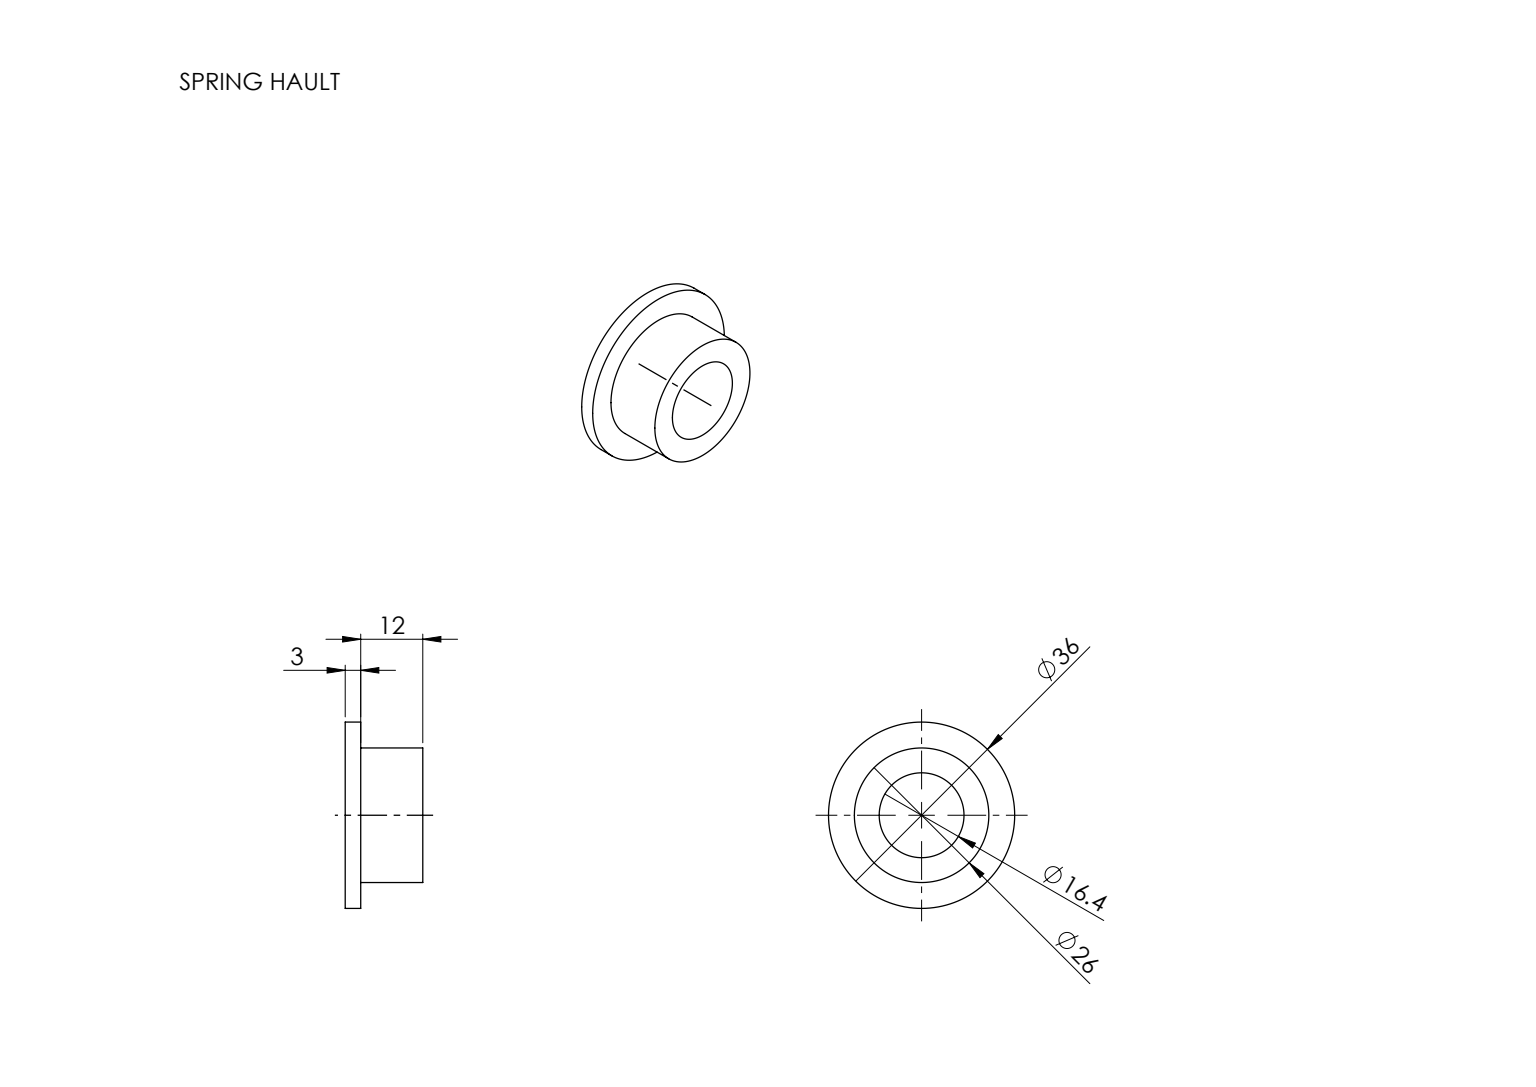
ISO-10303-21;
HEADER;
FILE_DESCRIPTION (('STEP AP214'),
    '1' );
FILE_NAME ('spring hault.step',
    '2026-10-08T13:22:57',
    ( '' ),
    ( '' ),
    'SwSTEP 2.0',
    'SolidWorks 2026',
    '' );
FILE_SCHEMA (( 'AUTOMOTIVE_DESIGN' ));
ENDSEC;

DATA;
#47=CIRCLE ( 'NONE', #69, 13.00000000000001066 ) ;
#65=ORIENTED_EDGE ( 'NONE', *, *, #5817, .F. ) ;
#69=AXIS2_PLACEMENT_3D ( 'NONE', #6608, #9795, #2698 ) ;
#113=( LENGTH_UNIT ( ) NAMED_UNIT ( * ) SI_UNIT ( .MILLI., .METRE. ) );
#143=ORIENTED_EDGE ( 'NONE', *, *, #7111, .T. ) ;
#157=CARTESIAN_POINT ( 'NONE',  ( -58.00000000000002842, 7.703719777548943412E-30, -1.059261469412979719E-30 ) ) ;
#169=CYLINDRICAL_SURFACE ( 'NONE', #4836, 18.00000000000002132 ) ;
#180=CIRCLE ( 'NONE', #1825, 18.00000000000002132 ) ;
#182=ORIENTED_EDGE ( 'NONE', *, *, #837, .T. ) ;
#193=UNCERTAINTY_MEASURE_WITH_UNIT (LENGTH_MEASURE( 1.000000000000000082E-05 ), #7498, 'distance_accuracy_value', 'NONE');
#203=VECTOR ( 'NONE', #8292, 1000.000000000000000 ) ;
#231=EDGE_CURVE ( 'NONE', #1952, #8798, #6117, .T. ) ;
#245=CARTESIAN_POINT ( 'NONE',  ( 0.000000000000000000, 0.000000000000000000, 0.000000000000000000 ) ) ;
#250=ORIENTED_EDGE ( 'NONE', *, *, #8801, .F. ) ;
#286=MANIFOLD_SOLID_BREP ( 'Revolve1', #1357 ) ;
#402=VECTOR ( 'NONE', #5225, 1000.000000000000000 ) ;
#433=EDGE_CURVE ( 'NONE', #9051, #3839, #8410, .T. ) ;
#459=AXIS2_PLACEMENT_3D ( 'NONE', #4903, #3979, #7954 ) ;
#490=CARTESIAN_POINT ( 'NONE',  ( -55.00000000000002132, 7.703719777548943412E-30, -7.703719777548943412E-31 ) ) ;
#571=EDGE_LOOP ( 'NONE', ( #1086, #3200, #2296, #1950 ) ) ;
#603=DIRECTION ( 'NONE',  ( -1.000000000000000000, 1.842239752758738928E-31, -1.780435181894459419E-32 ) ) ;
#626=FACE_OUTER_BOUND ( 'NONE', #2874, .T. ) ;
#649=CARTESIAN_POINT ( 'NONE',  ( -58.00000000000002842, 9.020562075080167263E-17, 13.00000000000001243 ) ) ;
#652=SURFACE_STYLE_FILL_AREA ( #4470 ) ;
#676=ORIENTED_EDGE ( 'NONE', *, *, #3604, .T. ) ;
#694=CYLINDRICAL_SURFACE ( 'NONE', #5832, 18.00000000000002132 ) ;
#707=PLANE ( 'NONE',  #2637 ) ;
#719=ADVANCED_FACE ( 'NONE', ( #7922, #8553 ), #707, .F. ) ;
#752=DIRECTION ( 'NONE',  ( -1.000000000000000000, 1.842239752758738928E-31, -1.780435181894459419E-32 ) ) ;
#795=ORIENTED_EDGE ( 'NONE', *, *, #5893, .F. ) ;
#837=EDGE_CURVE ( 'NONE', #7040, #4031, #8175, .T. ) ;
#849=CIRCLE ( 'NONE', #2646, 8.200000000000009948 ) ;
#863=EDGE_CURVE ( 'NONE', #8514, #4989, #4957, .T. ) ;
#991=FACE_OUTER_BOUND ( 'NONE', #5671, .T. ) ;
#1018=DIRECTION ( 'NONE',  ( 0.000000000000000000, 6.938893903907221444E-18, 1.000000000000000000 ) ) ;
#1021=COLOUR_RGB ( '', 0.72549020, 0.75294118, 0.79215686) ;
#1054=( NAMED_UNIT ( * ) SI_UNIT ( $, .STERADIAN. ) SOLID_ANGLE_UNIT ( ) );
#1073=DIRECTION ( 'NONE',  ( -1.000000000000000000, 1.842239752758738928E-31, -1.780435181894459419E-32 ) ) ;
#1086=ORIENTED_EDGE ( 'NONE', *, *, #4434, .F. ) ;
#1094=CARTESIAN_POINT ( 'NONE',  ( -58.00000000000002132, 5.689893001204698381E-17, 8.200000000000009948 ) ) ;
#1201=DIRECTION ( 'NONE',  ( -1.000000000000000000, 1.842239752758738928E-31, -1.780435181894459419E-32 ) ) ;
#1216=CARTESIAN_POINT ( 'NONE',  ( -43.00000000000002842, 6.933347799794049071E-30, -9.629649721936179265E-31 ) ) ;
#1224=AXIS2_PLACEMENT_3D ( 'NONE', #3055, #7082, #9483 ) ;
#1260=SURFACE_STYLE_USAGE ( .BOTH. , #3745 ) ;
#1297=ORIENTED_EDGE ( 'NONE', *, *, #6791, .F. ) ;
#1357=CLOSED_SHELL ( 'NONE', ( #6188, #6338, #4207, #6354, #4057, #6193, #3933, #5342, #719 ) ) ;
#1452=CARTESIAN_POINT ( 'NONE',  ( -55.00000000000002132, 18.00000000000001776, -1.819825643106760428E-16 ) ) ;
#1516=DIRECTION ( 'NONE',  ( 0.000000000000000000, 6.938893903907221444E-18, 1.000000000000000000 ) ) ;
#1660=EDGE_CURVE ( 'NONE', #7847, #3628, #10060, .T. ) ;
#1770=( NAMED_UNIT ( * ) PLANE_ANGLE_UNIT ( ) SI_UNIT ( $, .RADIAN. ) );
#1825=AXIS2_PLACEMENT_3D ( 'NONE', #3023, #603, #3749 ) ;
#1937=DIRECTION ( 'NONE',  ( -1.000000000000000000, 1.842239752758738928E-31, -1.780435181894459419E-32 ) ) ;
#1950=ORIENTED_EDGE ( 'NONE', *, *, #231, .F. ) ;
#1952=VERTEX_POINT ( 'NONE', #3909 ) ;
#2077=CARTESIAN_POINT ( 'NONE',  ( -58.00000000000002842, 2.079464148194916361E-15, -18.00000000000002132 ) ) ;
#2175=COLOUR_RGB ( '', 0.72549020, 0.75294118, 0.79215686) ;
#2178=PLANE ( 'NONE',  #459 ) ;
#2188=DIRECTION ( 'NONE',  ( -1.000000000000000000, 1.842239752758738928E-31, -1.780435181894459419E-32 ) ) ;
#2205=CARTESIAN_POINT ( 'NONE',  ( -43.00000000000002842, 5.689893001204620728E-17, 8.200000000000009948 ) ) ;
#2296=ORIENTED_EDGE ( 'NONE', *, *, #2974, .T. ) ;
#2301=DIRECTION ( 'NONE',  ( -1.840628461782073167E-32, -6.938893903907220674E-18, -1.000000000000000000 ) ) ;
#2308=ORIENTED_EDGE ( 'NONE', *, *, #5817, .T. ) ;
#2323=CIRCLE ( 'NONE', #9921, 18.00000000000001776 ) ;
#2350=CARTESIAN_POINT ( 'NONE',  ( -43.00000000000002842, 6.933347799794049071E-30, -9.629649721936179265E-31 ) ) ;
#2440=DIRECTION ( 'NONE',  ( 0.000000000000000000, 6.938893903907220674E-18, 1.000000000000000000 ) ) ;
#2478=ORIENTED_EDGE ( 'NONE', *, *, #2974, .F. ) ;
#2491=FILL_AREA_STYLE ('',( #7000 ) ) ;
#2525=DIRECTION ( 'NONE',  ( 0.000000000000000000, 6.938893903907220674E-18, 1.000000000000000000 ) ) ;
#2564=EDGE_CURVE ( 'NONE', #3839, #9051, #9098, .T. ) ;
#2574=ORIENTED_EDGE ( 'NONE', *, *, #4434, .T. ) ;
#2619=ORIENTED_EDGE ( 'NONE', *, *, #863, .F. ) ;
#2629=EDGE_LOOP ( 'NONE', ( #1297, #182, #3115, #7849 ) ) ;
#2637=AXIS2_PLACEMENT_3D ( 'NONE', #6994, #3069, #2301 ) ;
#2646=AXIS2_PLACEMENT_3D ( 'NONE', #1216, #6571, #9806 ) ;
#2698=DIRECTION ( 'NONE',  ( 0.000000000000000000, 6.938893903907221444E-18, 1.000000000000000000 ) ) ;
#2718=ORIENTED_EDGE ( 'NONE', *, *, #1660, .T. ) ;
#2725=PRODUCT_CONTEXT ( 'NONE', #5533, 'mechanical' ) ;
#2742=AXIS2_PLACEMENT_3D ( 'NONE', #7490, #8319, #5061 ) ;
#2808=( NAMED_UNIT ( * ) SI_UNIT ( $, .STERADIAN. ) SOLID_ANGLE_UNIT ( ) );
#2842=AXIS2_PLACEMENT_3D ( 'NONE', #3609, #6028, #9208 ) ;
#2859=( NAMED_UNIT ( * ) PLANE_ANGLE_UNIT ( ) SI_UNIT ( $, .RADIAN. ) );
#2874=EDGE_LOOP ( 'NONE', ( #5790, #7225 ) ) ;
#2883=CARTESIAN_POINT ( 'NONE',  ( -43.00000000000002842, 1.501835218140771832E-15, -13.00000000000000178 ) ) ;
#2974=EDGE_CURVE ( 'NONE', #9051, #8798, #8703, .T. ) ;
#3023=CARTESIAN_POINT ( 'NONE',  ( -58.00000000000002132, 7.703719777548943412E-30, -1.059261469412979719E-30 ) ) ;
#3042=VERTEX_POINT ( 'NONE', #5497 ) ;
#3055=CARTESIAN_POINT ( 'NONE',  ( -58.00000000000002842, 7.703719777548943412E-30, -1.059261469412979719E-30 ) ) ;
#3069=DIRECTION ( 'NONE',  ( 1.000000000000000000, -1.842239752758738928E-31, -1.840628461782073167E-32 ) ) ;
#3115=ORIENTED_EDGE ( 'NONE', *, *, #5908, .T. ) ;
#3165=CARTESIAN_POINT ( 'NONE',  ( -43.00000000000002842, 9.020562075080090842E-17, 13.00000000000001421 ) ) ;
#3200=ORIENTED_EDGE ( 'NONE', *, *, #2564, .T. ) ;
#3211=ORIENTED_EDGE ( 'NONE', *, *, #7111, .F. ) ;
#3221=ORIENTED_EDGE ( 'NONE', *, *, #433, .T. ) ;
#3256=EDGE_LOOP ( 'NONE', ( #10227, #8788, #8586, #3337 ) ) ;
#3259=CARTESIAN_POINT ( 'NONE',  ( -58.00000000000002842, 7.703719777548943412E-30, -1.059261469412979719E-30 ) ) ;
#3279=EDGE_LOOP ( 'NONE', ( #143, #4180 ) ) ;
#3323=SURFACE_STYLE_USAGE ( .BOTH. , #8018 ) ;
#3337=ORIENTED_EDGE ( 'NONE', *, *, #8669, .F. ) ;
#3369=AXIS2_PLACEMENT_3D ( 'NONE', #8279, #1201, #8330 ) ;
#3422=CARTESIAN_POINT ( 'NONE',  ( -58.00000000000002132, 7.703719777548943412E-30, -1.059261469412979719E-30 ) ) ;
#3464=( NAMED_UNIT ( * ) SI_UNIT ( $, .STERADIAN. ) SOLID_ANGLE_UNIT ( ) );
#3525=PRODUCT ( 'spring hault', 'spring hault', '', ( #2725 ) ) ;
#3604=EDGE_CURVE ( 'NONE', #9714, #3042, #4405, .T. ) ;
#3609=CARTESIAN_POINT ( 'NONE',  ( -43.00000000000002842, 6.933347799794049071E-30, -9.629649721936179265E-31 ) ) ;
#3628=VERTEX_POINT ( 'NONE', #1094 ) ;
#3629=ADVANCED_BREP_SHAPE_REPRESENTATION ( '', ( #286, #3995 ), #5470 ) ;
#3653=STYLED_ITEM ( 'NONE', ( #4148 ), #3629 ) ;
#3664=DIRECTION ( 'NONE',  ( 1.840628461782073167E-32, 6.938893903907220674E-18, 1.000000000000000000 ) ) ;
#3675=( NAMED_UNIT ( * ) PLANE_ANGLE_UNIT ( ) SI_UNIT ( $, .RADIAN. ) );
#3717=CARTESIAN_POINT ( 'NONE',  ( -58.00000000000002132, 9.473114452887969885E-16, -8.200000000000001066 ) ) ;
#3745=SURFACE_SIDE_STYLE ('',( #652 ) ) ;
#3749=DIRECTION ( 'NONE',  ( 0.000000000000000000, 6.938893903907221444E-18, 1.000000000000000000 ) ) ;
#3801=( GEOMETRIC_REPRESENTATION_CONTEXT ( 3 ) GLOBAL_UNCERTAINTY_ASSIGNED_CONTEXT ( ( #8778 ) ) GLOBAL_UNIT_ASSIGNED_CONTEXT ( ( #6881, #2859, #2808 ) ) REPRESENTATION_CONTEXT ( 'NONE', 'WORKASPACE' ) );
#3810=AXIS2_PLACEMENT_3D ( 'NONE', #6405, #4922, #2440 ) ;
#3839=VERTEX_POINT ( 'NONE', #2883 ) ;
#3854=DIRECTION ( 'NONE',  ( -1.000000000000000000, 1.842239752758738928E-31, -1.780435181894459419E-32 ) ) ;
#3909=CARTESIAN_POINT ( 'NONE',  ( -55.00000000000002132, 1.501835218140771437E-15, -12.99999999999999822 ) ) ;
#3933=ADVANCED_FACE ( 'NONE', ( #626, #5370 ), #8634, .F. ) ;
#3979=DIRECTION ( 'NONE',  ( -1.000000000000000000, 1.842239752758738928E-31, 1.840628461782073167E-32 ) ) ;
#3994=FACE_OUTER_BOUND ( 'NONE', #10023, .T. ) ;
#3995=AXIS2_PLACEMENT_3D ( 'NONE', #245, #8930, #7419 ) ;
#4031=VERTEX_POINT ( 'NONE', #3717 ) ;
#4057=ADVANCED_FACE ( 'NONE', ( #6078, #9256 ), #2178, .F. ) ;
#4148=PRESENTATION_STYLE_ASSIGNMENT (( #3323 ) ) ;
#4180=ORIENTED_EDGE ( 'NONE', *, *, #6791, .T. ) ;
#4207=ADVANCED_FACE ( 'NONE', ( #4754 ), #9623, .F. ) ;
#4405=CIRCLE ( 'NONE', #2742, 18.00000000000001776 ) ;
#4419=DIRECTION ( 'NONE',  ( 0.000000000000000000, 6.938893903907221444E-18, 1.000000000000000000 ) ) ;
#4434=EDGE_CURVE ( 'NONE', #3839, #1952, #6052, .T. ) ;
#4470=FILL_AREA_STYLE ('',( #8293 ) ) ;
#4507=CARTESIAN_POINT ( 'NONE',  ( -55.00000000000002132, 2.079464148194913206E-15, -18.00000000000000000 ) ) ;
#4626=DIRECTION ( 'NONE',  ( 0.000000000000000000, 6.938893903907221444E-18, 1.000000000000000000 ) ) ;
#4634=VECTOR ( 'NONE', #9964, 1000.000000000000000 ) ;
#4702=DIRECTION ( 'NONE',  ( -1.000000000000000000, 1.842239752758738928E-31, 1.840628461782073167E-32 ) ) ;
#4742=PRODUCT_DEFINITION_CONTEXT ( 'detailed design', #7509, 'design' ) ;
#4754=FACE_OUTER_BOUND ( 'NONE', #2629, .T. ) ;
#4768=DIRECTION ( 'NONE',  ( -1.000000000000000000, 1.842239752758738928E-31, -1.780435181894459419E-32 ) ) ;
#4836=AXIS2_PLACEMENT_3D ( 'NONE', #4879, #7401, #5029 ) ;
#4853=CARTESIAN_POINT ( 'NONE',  ( -58.00000000000002842, 7.703719777548943412E-30, -1.059261469412979719E-30 ) ) ;
#4879=CARTESIAN_POINT ( 'NONE',  ( -58.00000000000002842, 7.703719777548943412E-30, -1.059261469412979719E-30 ) ) ;
#4903=CARTESIAN_POINT ( 'NONE',  ( -43.00000000000002842, 8.200000000000018829, 8.906797881070005341E-17 ) ) ;
#4922=DIRECTION ( 'NONE',  ( -1.000000000000000000, 1.842239752758738928E-31, -1.780435181894459419E-32 ) ) ;
#4957=CIRCLE ( 'NONE', #6430, 18.00000000000002132 ) ;
#4989=VERTEX_POINT ( 'NONE', #9387 ) ;
#5029=DIRECTION ( 'NONE',  ( 0.000000000000000000, 6.938893903907221444E-18, 1.000000000000000000 ) ) ;
#5061=DIRECTION ( 'NONE',  ( 0.000000000000000000, 6.938893903907221444E-18, 1.000000000000000000 ) ) ;
#5128=LINE ( 'NONE', #2077, #402 ) ;
#5147=UNCERTAINTY_MEASURE_WITH_UNIT (LENGTH_MEASURE( 1.000000000000000082E-05 ), #113, 'distance_accuracy_value', 'NONE');
#5195=CARTESIAN_POINT ( 'NONE',  ( -55.00000000000002132, 7.703719777548943412E-30, -7.703719777548943412E-31 ) ) ;
#5225=DIRECTION ( 'NONE',  ( -1.000000000000000000, 1.842239752758738928E-31, -1.780435181894459419E-32 ) ) ;
#5342=ADVANCED_FACE ( 'NONE', ( #7248 ), #169, .T. ) ;
#5370=FACE_BOUND ( 'NONE', #5472, .T. ) ;
#5417=PRODUCT_DEFINITION_FORMATION_WITH_SPECIFIED_SOURCE ( 'ANY', '', #3525, .NOT_KNOWN. ) ;
#5470=( GEOMETRIC_REPRESENTATION_CONTEXT ( 3 ) GLOBAL_UNCERTAINTY_ASSIGNED_CONTEXT ( ( #5147 ) ) GLOBAL_UNIT_ASSIGNED_CONTEXT ( ( #113, #1770, #1054 ) ) REPRESENTATION_CONTEXT ( 'NONE', 'WORKASPACE' ) );
#5472=EDGE_LOOP ( 'NONE', ( #2308, #6066 ) ) ;
#5489=FACE_OUTER_BOUND ( 'NONE', #3256, .T. ) ;
#5497=CARTESIAN_POINT ( 'NONE',  ( -55.00000000000002132, 1.249000902703378022E-16, 18.00000000000001776 ) ) ;
#5533=APPLICATION_CONTEXT ( 'automotive_design' ) ;
#5640=LINE ( 'NONE', #7193, #8427 ) ;
#5642=SURFACE_STYLE_FILL_AREA ( #2491 ) ;
#5671=EDGE_LOOP ( 'NONE', ( #7619, #3211, #2718, #5801 ) ) ;
#5675=CIRCLE ( 'NONE', #3369, 8.200000000000009948 ) ;
#5695=DIRECTION ( 'NONE',  ( 0.000000000000000000, 6.938893903907221444E-18, 1.000000000000000000 ) ) ;
#5727=AXIS2_PLACEMENT_3D ( 'NONE', #1452, #4702, #3664 ) ;
#5790=ORIENTED_EDGE ( 'NONE', *, *, #7151, .F. ) ;
#5801=ORIENTED_EDGE ( 'NONE', *, *, #8801, .T. ) ;
#5817=EDGE_CURVE ( 'NONE', #8798, #1952, #47, .T. ) ;
#5832=AXIS2_PLACEMENT_3D ( 'NONE', #10141, #2188, #1516 ) ;
#5893=EDGE_CURVE ( 'NONE', #9714, #8514, #5128, .T. ) ;
#5908=EDGE_CURVE ( 'NONE', #4031, #3628, #5675, .T. ) ;
#5934=AXIS2_PLACEMENT_3D ( 'NONE', #9026, #1937, #9131 ) ;
#5954=CARTESIAN_POINT ( 'NONE',  ( -58.00000000000002842, 1.501835218140774790E-15, -13.00000000000001243 ) ) ;
#6028=DIRECTION ( 'NONE',  ( -1.000000000000000000, 1.842239752758738928E-31, -1.780435181894459419E-32 ) ) ;
#6052=LINE ( 'NONE', #5954, #203 ) ;
#6066=ORIENTED_EDGE ( 'NONE', *, *, #231, .T. ) ;
#6078=FACE_OUTER_BOUND ( 'NONE', #9586, .T. ) ;
#6117=CIRCLE ( 'NONE', #6602, 13.00000000000001066 ) ;
#6188=ADVANCED_FACE ( 'NONE', ( #5489 ), #694, .T. ) ;
#6193=ADVANCED_FACE ( 'NONE', ( #8646 ), #10091, .T. ) ;
#6326=CIRCLE ( 'NONE', #2842, 8.200000000000009948 ) ;
#6338=ADVANCED_FACE ( 'NONE', ( #3994 ), #7238, .T. ) ;
#6354=ADVANCED_FACE ( 'NONE', ( #991 ), #6499, .F. ) ;
#6387=ORIENTED_EDGE ( 'NONE', *, *, #7867, .T. ) ;
#6401=DIRECTION ( 'NONE',  ( 0.000000000000000000, 6.938893903907220674E-18, 1.000000000000000000 ) ) ;
#6405=CARTESIAN_POINT ( 'NONE',  ( -58.00000000000002132, 7.703719777548943412E-30, -1.059261469412979719E-30 ) ) ;
#6422=STYLED_ITEM ( 'NONE', ( #6770 ), #286 ) ;
#6430=AXIS2_PLACEMENT_3D ( 'NONE', #3422, #6560, #5695 ) ;
#6453=DIRECTION ( 'NONE',  ( -1.000000000000000000, 1.842239752758738928E-31, -1.780435181894459419E-32 ) ) ;
#6499=CYLINDRICAL_SURFACE ( 'NONE', #7489, 8.200000000000009948 ) ;
#6552=PRODUCT_DEFINITION_SHAPE ( 'NONE', 'NONE',  #6660 ) ;
#6560=DIRECTION ( 'NONE',  ( -1.000000000000000000, 1.842239752758738928E-31, -1.780435181894459419E-32 ) ) ;
#6571=DIRECTION ( 'NONE',  ( -1.000000000000000000, 1.842239752758738928E-31, -1.780435181894459419E-32 ) ) ;
#6602=AXIS2_PLACEMENT_3D ( 'NONE', #490, #10050, #4419 ) ;
#6608=CARTESIAN_POINT ( 'NONE',  ( -55.00000000000002132, 7.703719777548943412E-30, -7.703719777548943412E-31 ) ) ;
#6660=PRODUCT_DEFINITION ( 'UNKNOWN', '', #5417, #4742 ) ;
#6676=CARTESIAN_POINT ( 'NONE',  ( -58.00000000000002842, 5.689893001204698381E-17, 8.200000000000009948 ) ) ;
#6687=VECTOR ( 'NONE', #752, 1000.000000000000000 ) ;
#6770=PRESENTATION_STYLE_ASSIGNMENT (( #1260 ) ) ;
#6778=AXIS2_PLACEMENT_3D ( 'NONE', #4853, #7280, #2525 ) ;
#6791=EDGE_CURVE ( 'NONE', #7040, #7847, #6326, .T. ) ;
#6881=( LENGTH_UNIT ( ) NAMED_UNIT ( * ) SI_UNIT ( .MILLI., .METRE. ) );
#6983=CARTESIAN_POINT ( 'NONE',  ( -58.00000000000002132, 2.079464148194913600E-15, -18.00000000000000355 ) ) ;
#6994=CARTESIAN_POINT ( 'NONE',  ( -58.00000000000002132, 8.200000000000009948, 5.769589564291770364E-16 ) ) ;
#7000=FILL_AREA_STYLE_COLOUR ( '', #1021 ) ;
#7040=VERTEX_POINT ( 'NONE', #7938 ) ;
#7079=ORIENTED_EDGE ( 'NONE', *, *, #8669, .T. ) ;
#7082=DIRECTION ( 'NONE',  ( -1.000000000000000000, 1.842239752758738928E-31, -1.780435181894459419E-32 ) ) ;
#7111=EDGE_CURVE ( 'NONE', #7847, #7040, #849, .T. ) ;
#7151=EDGE_CURVE ( 'NONE', #3042, #9714, #2323, .T. ) ;
#7165=AXIS2_PLACEMENT_3D ( 'NONE', #157, #6453, #8063 ) ;
#7190=DIRECTION ( 'NONE',  ( -1.000000000000000000, 1.842239752758738928E-31, -1.780435181894459419E-32 ) ) ;
#7193=CARTESIAN_POINT ( 'NONE',  ( -58.00000000000002842, 1.249000902703378268E-16, 18.00000000000002132 ) ) ;
#7225=ORIENTED_EDGE ( 'NONE', *, *, #3604, .F. ) ;
#7238=CYLINDRICAL_SURFACE ( 'NONE', #7165, 13.00000000000001243 ) ;
#7248=FACE_OUTER_BOUND ( 'NONE', #8416, .T. ) ;
#7280=DIRECTION ( 'NONE',  ( -1.000000000000000000, 1.842239752758738928E-31, -1.780435181894459419E-32 ) ) ;
#7303=DIRECTION ( 'NONE',  ( -1.000000000000000000, 1.842239752758738928E-31, -1.780435181894459419E-32 ) ) ;
#7361=ORIENTED_EDGE ( 'NONE', *, *, #433, .F. ) ;
#7401=DIRECTION ( 'NONE',  ( -1.000000000000000000, 1.842239752758738928E-31, -1.780435181894459419E-32 ) ) ;
#7419=DIRECTION ( 'NONE',  ( 1.000000000000000000, 0.000000000000000000, 0.000000000000000000 ) ) ;
#7489=AXIS2_PLACEMENT_3D ( 'NONE', #3259, #7190, #6401 ) ;
#7490=CARTESIAN_POINT ( 'NONE',  ( -55.00000000000002132, 7.703719777548943412E-30, -7.703719777548943412E-31 ) ) ;
#7498=( LENGTH_UNIT ( ) NAMED_UNIT ( * ) SI_UNIT ( .MILLI., .METRE. ) );
#7509=APPLICATION_CONTEXT ( 'automotive_design' ) ;
#7604=CIRCLE ( 'NONE', #3810, 8.200000000000009948 ) ;
#7619=ORIENTED_EDGE ( 'NONE', *, *, #837, .F. ) ;
#7764=VECTOR ( 'NONE', #7303, 1000.000000000000000 ) ;
#7847=VERTEX_POINT ( 'NONE', #2205 ) ;
#7849=ORIENTED_EDGE ( 'NONE', *, *, #1660, .F. ) ;
#7867=EDGE_CURVE ( 'NONE', #4989, #8514, #180, .T. ) ;
#7896=EDGE_LOOP ( 'NONE', ( #250, #10126 ) ) ;
#7916=AXIS2_PLACEMENT_3D ( 'NONE', #2350, #3854, #4626 ) ;
#7922=FACE_BOUND ( 'NONE', #7896, .T. ) ;
#7938=CARTESIAN_POINT ( 'NONE',  ( -43.00000000000002842, 9.473114452887969885E-16, -8.200000000000001066 ) ) ;
#7954=DIRECTION ( 'NONE',  ( 1.840628461782073167E-32, 6.938893903907220674E-18, 1.000000000000000000 ) ) ;
#8018=SURFACE_SIDE_STYLE ('',( #5642 ) ) ;
#8059=EDGE_LOOP ( 'NONE', ( #6387, #9965 ) ) ;
#8063=DIRECTION ( 'NONE',  ( 0.000000000000000000, 6.938893903907221444E-18, 1.000000000000000000 ) ) ;
#8175=LINE ( 'NONE', #8863, #7764 ) ;
#8217=SHAPE_REPRESENTATION_RELATIONSHIP ( 'NONE' , 'NONE' ,  #10217, #3629 ) ;
#8257=SHAPE_DEFINITION_REPRESENTATION ( #6552, #10217 ) ;
#8279=CARTESIAN_POINT ( 'NONE',  ( -58.00000000000002132, 7.703719777548943412E-30, -1.059261469412979719E-30 ) ) ;
#8292=DIRECTION ( 'NONE',  ( -1.000000000000000000, 1.842239752758738928E-31, -1.780435181894459419E-32 ) ) ;
#8293=FILL_AREA_STYLE_COLOUR ( '', #2175 ) ;
#8319=DIRECTION ( 'NONE',  ( -1.000000000000000000, 1.842239752758738928E-31, -1.780435181894459419E-32 ) ) ;
#8330=DIRECTION ( 'NONE',  ( 0.000000000000000000, 6.938893903907220674E-18, 1.000000000000000000 ) ) ;
#8410=CIRCLE ( 'NONE', #7916, 13.00000000000001421 ) ;
#8416=EDGE_LOOP ( 'NONE', ( #795, #676, #7079, #2619 ) ) ;
#8427=VECTOR ( 'NONE', #4768, 1000.000000000000000 ) ;
#8514=VERTEX_POINT ( 'NONE', #6983 ) ;
#8553=FACE_OUTER_BOUND ( 'NONE', #8059, .T. ) ;
#8586=ORIENTED_EDGE ( 'NONE', *, *, #7867, .F. ) ;
#8634=PLANE ( 'NONE',  #5727 ) ;
#8646=FACE_OUTER_BOUND ( 'NONE', #571, .T. ) ;
#8669=EDGE_CURVE ( 'NONE', #3042, #4989, #5640, .T. ) ;
#8703=LINE ( 'NONE', #649, #6687 ) ;
#8747=CARTESIAN_POINT ( 'NONE',  ( -55.00000000000002132, 9.020562075080166030E-17, 13.00000000000001066 ) ) ;
#8778=UNCERTAINTY_MEASURE_WITH_UNIT (LENGTH_MEASURE( 1.000000000000000082E-05 ), #6881, 'distance_accuracy_value', 'NONE');
#8786=( GEOMETRIC_REPRESENTATION_CONTEXT ( 3 ) GLOBAL_UNCERTAINTY_ASSIGNED_CONTEXT ( ( #193 ) ) GLOBAL_UNIT_ASSIGNED_CONTEXT ( ( #7498, #3675, #3464 ) ) REPRESENTATION_CONTEXT ( 'NONE', 'WORKASPACE' ) );
#8788=ORIENTED_EDGE ( 'NONE', *, *, #5893, .T. ) ;
#8798=VERTEX_POINT ( 'NONE', #8747 ) ;
#8801=EDGE_CURVE ( 'NONE', #3628, #4031, #7604, .T. ) ;
#8863=CARTESIAN_POINT ( 'NONE',  ( -58.00000000000002842, 9.473114452887993551E-16, -8.200000000000009948 ) ) ;
#8930=DIRECTION ( 'NONE',  ( 0.000000000000000000, 0.000000000000000000, 1.000000000000000000 ) ) ;
#9026=CARTESIAN_POINT ( 'NONE',  ( -43.00000000000002842, 6.933347799794049071E-30, -9.629649721936179265E-31 ) ) ;
#9051=VERTEX_POINT ( 'NONE', #3165 ) ;
#9098=CIRCLE ( 'NONE', #5934, 13.00000000000001421 ) ;
#9131=DIRECTION ( 'NONE',  ( 0.000000000000000000, 6.938893903907221444E-18, 1.000000000000000000 ) ) ;
#9208=DIRECTION ( 'NONE',  ( 0.000000000000000000, 6.938893903907220674E-18, 1.000000000000000000 ) ) ;
#9256=FACE_BOUND ( 'NONE', #3279, .T. ) ;
#9274=MECHANICAL_DESIGN_GEOMETRIC_PRESENTATION_REPRESENTATION('',(#6422),#3801);
#9387=CARTESIAN_POINT ( 'NONE',  ( -58.00000000000002132, 1.249000902703378268E-16, 18.00000000000002132 ) ) ;
#9450=MECHANICAL_DESIGN_GEOMETRIC_PRESENTATION_REPRESENTATION('',(#3653),#8786);
#9483=DIRECTION ( 'NONE',  ( 0.000000000000000000, 6.938893903907221444E-18, 1.000000000000000000 ) ) ;
#9586=EDGE_LOOP ( 'NONE', ( #7361, #10011 ) ) ;
#9623=CYLINDRICAL_SURFACE ( 'NONE', #6778, 8.200000000000009948 ) ;
#9714=VERTEX_POINT ( 'NONE', #4507 ) ;
#9795=DIRECTION ( 'NONE',  ( -1.000000000000000000, 1.842239752758738928E-31, -1.780435181894459419E-32 ) ) ;
#9806=DIRECTION ( 'NONE',  ( 0.000000000000000000, 6.938893903907220674E-18, 1.000000000000000000 ) ) ;
#9921=AXIS2_PLACEMENT_3D ( 'NONE', #5195, #1073, #1018 ) ;
#9964=DIRECTION ( 'NONE',  ( -1.000000000000000000, 1.842239752758738928E-31, -1.780435181894459419E-32 ) ) ;
#9965=ORIENTED_EDGE ( 'NONE', *, *, #863, .T. ) ;
#10011=ORIENTED_EDGE ( 'NONE', *, *, #2564, .F. ) ;
#10023=EDGE_LOOP ( 'NONE', ( #3221, #2574, #65, #2478 ) ) ;
#10050=DIRECTION ( 'NONE',  ( -1.000000000000000000, 1.842239752758738928E-31, -1.780435181894459419E-32 ) ) ;
#10060=LINE ( 'NONE', #6676, #4634 ) ;
#10091=CYLINDRICAL_SURFACE ( 'NONE', #1224, 13.00000000000001243 ) ;
#10126=ORIENTED_EDGE ( 'NONE', *, *, #5908, .F. ) ;
#10141=CARTESIAN_POINT ( 'NONE',  ( -58.00000000000002842, 7.703719777548943412E-30, -1.059261469412979719E-30 ) ) ;
#10217=SHAPE_REPRESENTATION ( 'spring hault', ( #3995 ), #5470 ) ;
#10227=ORIENTED_EDGE ( 'NONE', *, *, #7151, .T. ) ;
ENDSEC;
END-ISO-10303-21;
